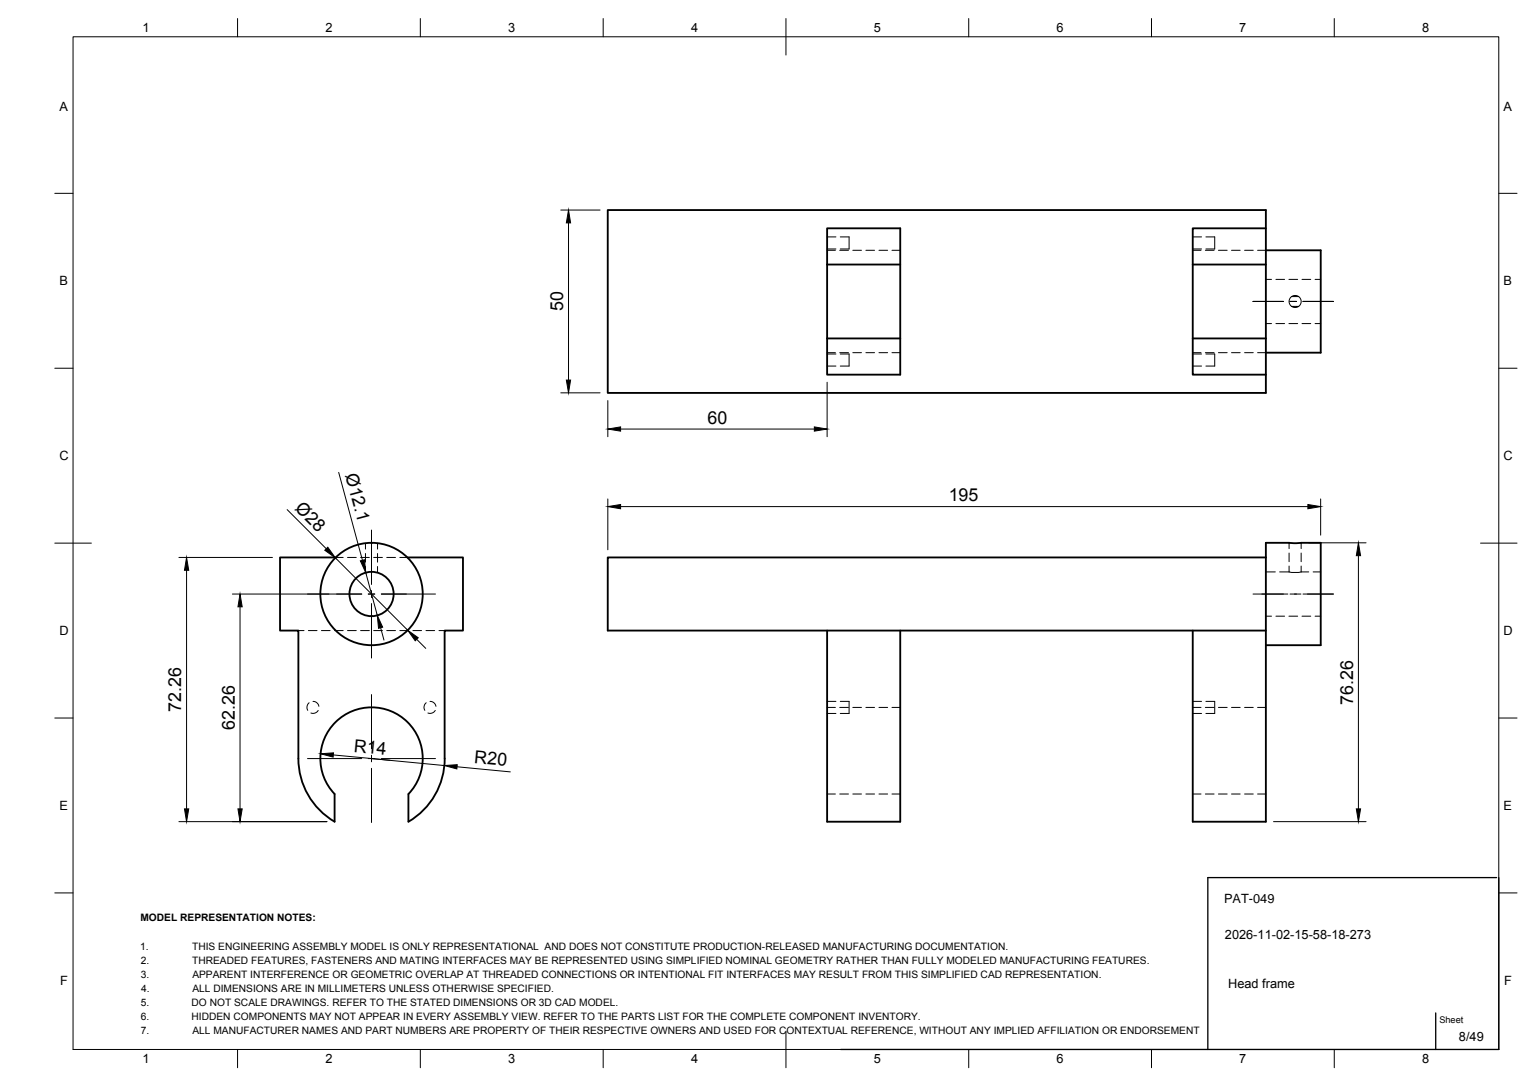
ISO-10303-21;
HEADER;
/* Generated by software containing ST-Developer
 * from STEP Tools, Inc. (www.steptools.com) 
 */

FILE_DESCRIPTION(
/* description */ ('Hand drill press frame (manual)'),
/* implementation_level */ '2;1');

FILE_NAME(
/* name */ 'Head frame.step',
/* time_stamp */ '2026-10-28T03:25:28-07:00',
/* author */ (''),
/* organization */ (''),
/* preprocessor_version */ 'ST-DEVELOPER v20.2',
/* originating_system */ 'Autodesk Translation Framework v15.17.0.0',
/* authorisation */ '');

FILE_SCHEMA (('AUTOMOTIVE_DESIGN { 1 0 10303 214 3 1 1 }'));
ENDSEC;

DATA;
#10=MECHANICAL_DESIGN_GEOMETRIC_PRESENTATION_REPRESENTATION('',(#622),#33299);
#491=B_SPLINE_CURVE_WITH_KNOTS('',3,(#18163,#18164,#18165,#18166,#18167,
#18168,#18169,#18170,#18171,#18172,#18173,#18174,#18175,#18176),
 .UNSPECIFIED.,.F.,.F.,(4,2,2,2,2,2,4),(0.598759573717645,0.624973342427789,
0.687463163426141,0.749952984424493,0.812442805422845,0.874932626421197,
0.901146395131337),.UNSPECIFIED.);
#492=B_SPLINE_CURVE_WITH_KNOTS('',3,(#18180,#18181,#18182,#18183,#18184,
#18185,#18186,#18187),.UNSPECIFIED.,.F.,.F.,(4,2,2,4),(0.249984328141498,
0.31247414913985,0.374963970138202,0.401177738848345),.UNSPECIFIED.);
#493=B_SPLINE_CURVE_WITH_KNOTS('',3,(#18191,#18192,#18193,#18194,#18195,
#18196,#18197,#18198,#18199,#18200,#18201,#18202,#18203,#18204,#18205,#18206,
#18207,#18208,#18209,#18210,#18211,#18212,#18213,#18214,#18215,#18216),
 .UNSPECIFIED.,.F.,.F.,(4,2,2,2,2,2,2,2,2,2,2,2,4),(0.,0.0622156192199746,
0.124431238439949,0.186646447577113,0.248861656714277,0.31107686585144,
0.373292074988604,0.435507694208579,0.497723313428553,0.559938932648528,
0.622154551868502,0.684369761005666,0.74658497014283),.UNSPECIFIED.);
#494=B_SPLINE_CURVE_WITH_KNOTS('',3,(#18217,#18218,#18219,#18220,#18221,
#18222,#18223,#18224,#18225,#18226),.UNSPECIFIED.,.F.,.F.,(4,2,2,2,4),(0.74658497014283,
0.808800179279993,0.871015388417157,0.933231007637132,0.995446626857106),
 .UNSPECIFIED.);
#495=B_SPLINE_CURVE_WITH_KNOTS('',3,(#18227,#18228,#18229,#18230,#18231,
#18232,#18233,#18234),.UNSPECIFIED.,.F.,.F.,(4,2,2,4),(0.098790917434652,
0.125004686144793,0.187494507143146,0.249984328141498),.UNSPECIFIED.);
#532=SHAPE_REPRESENTATION_RELATIONSHIP('SRR','None',#33491,#577);
#577=ADVANCED_BREP_SHAPE_REPRESENTATION('',(#674),#33253);
#622=STYLED_ITEM('',(#33793),#674);
#674=MANIFOLD_SOLID_BREP('Body1',#12640);
#732=FACE_BOUND('',#2075,.T.);
#733=FACE_BOUND('',#2076,.T.);
#734=FACE_BOUND('',#2090,.T.);
#735=FACE_BOUND('',#2091,.T.);
#736=FACE_BOUND('',#2095,.T.);
#737=FACE_BOUND('',#2101,.T.);
#738=FACE_BOUND('',#2103,.T.);
#739=FACE_BOUND('',#2105,.T.);
#905=PLANE('',#13233);
#906=PLANE('',#13237);
#907=PLANE('',#13238);
#908=PLANE('',#13239);
#909=PLANE('',#13240);
#910=PLANE('',#13250);
#911=PLANE('',#13251);
#912=PLANE('',#13252);
#913=PLANE('',#13256);
#914=PLANE('',#13260);
#915=PLANE('',#13261);
#916=PLANE('',#13262);
#917=PLANE('',#13263);
#918=PLANE('',#13275);
#919=PLANE('',#13276);
#920=PLANE('',#13277);
#921=PLANE('',#13278);
#922=PLANE('',#13279);
#923=PLANE('',#13283);
#924=PLANE('',#13284);
#925=PLANE('',#13291);
#926=PLANE('',#13292);
#927=PLANE('',#13293);
#928=PLANE('',#13294);
#929=PLANE('',#13295);
#930=PLANE('',#13296);
#1363=FACE_OUTER_BOUND('',#2064,.T.);
#1364=FACE_OUTER_BOUND('',#2065,.T.);
#1365=FACE_OUTER_BOUND('',#2066,.T.);
#1366=FACE_OUTER_BOUND('',#2067,.T.);
#1367=FACE_OUTER_BOUND('',#2068,.T.);
#1368=FACE_OUTER_BOUND('',#2069,.T.);
#1369=FACE_OUTER_BOUND('',#2070,.T.);
#1370=FACE_OUTER_BOUND('',#2071,.T.);
#1371=FACE_OUTER_BOUND('',#2072,.T.);
#1372=FACE_OUTER_BOUND('',#2073,.T.);
#1373=FACE_OUTER_BOUND('',#2074,.T.);
#1374=FACE_OUTER_BOUND('',#2077,.T.);
#1375=FACE_OUTER_BOUND('',#2078,.T.);
#1376=FACE_OUTER_BOUND('',#2079,.T.);
#1377=FACE_OUTER_BOUND('',#2080,.T.);
#1378=FACE_OUTER_BOUND('',#2081,.T.);
#1379=FACE_OUTER_BOUND('',#2082,.T.);
#1380=FACE_OUTER_BOUND('',#2083,.T.);
#1381=FACE_OUTER_BOUND('',#2084,.T.);
#1382=FACE_OUTER_BOUND('',#2085,.T.);
#1383=FACE_OUTER_BOUND('',#2086,.T.);
#1384=FACE_OUTER_BOUND('',#2087,.T.);
#1385=FACE_OUTER_BOUND('',#2088,.T.);
#1386=FACE_OUTER_BOUND('',#2089,.T.);
#1387=FACE_OUTER_BOUND('',#2092,.T.);
#1388=FACE_OUTER_BOUND('',#2093,.T.);
#1389=FACE_OUTER_BOUND('',#2094,.T.);
#1390=FACE_OUTER_BOUND('',#2096,.T.);
#1391=FACE_OUTER_BOUND('',#2097,.T.);
#1392=FACE_OUTER_BOUND('',#2098,.T.);
#1393=FACE_OUTER_BOUND('',#2099,.T.);
#1394=FACE_OUTER_BOUND('',#2100,.T.);
#1395=FACE_OUTER_BOUND('',#2102,.T.);
#1396=FACE_OUTER_BOUND('',#2104,.T.);
#1397=FACE_OUTER_BOUND('',#2106,.T.);
#1398=FACE_OUTER_BOUND('',#2107,.T.);
#1399=FACE_OUTER_BOUND('',#2108,.T.);
#1400=FACE_OUTER_BOUND('',#2109,.T.);
#1401=FACE_OUTER_BOUND('',#2110,.T.);
#2064=EDGE_LOOP('',(#8529,#8530,#8531,#8532));
#2065=EDGE_LOOP('',(#8533));
#2066=EDGE_LOOP('',(#8534,#8535,#8536,#8537));
#2067=EDGE_LOOP('',(#8538));
#2068=EDGE_LOOP('',(#8539,#8540,#8541,#8542));
#2069=EDGE_LOOP('',(#8543,#8544,#8545,#8546));
#2070=EDGE_LOOP('',(#8547,#8548,#8549,#8550,#8551,#8552,#8553,#8554));
#2071=EDGE_LOOP('',(#8555,#8556,#8557,#8558));
#2072=EDGE_LOOP('',(#8559,#8560,#8561,#8562));
#2073=EDGE_LOOP('',(#8563,#8564,#8565,#8566));
#2074=EDGE_LOOP('',(#8567,#8568,#8569,#8570,#8571,#8572,#8573,#8574));
#2075=EDGE_LOOP('',(#8575));
#2076=EDGE_LOOP('',(#8576));
#2077=EDGE_LOOP('',(#8577,#8578,#8579,#8580));
#2078=EDGE_LOOP('',(#8581,#8582,#8583,#8584));
#2079=EDGE_LOOP('',(#8585,#8586,#8587,#8588));
#2080=EDGE_LOOP('',(#8589));
#2081=EDGE_LOOP('',(#8590,#8591,#8592,#8593));
#2082=EDGE_LOOP('',(#8594));
#2083=EDGE_LOOP('',(#8595,#8596,#8597,#8598));
#2084=EDGE_LOOP('',(#8599,#8600,#8601,#8602));
#2085=EDGE_LOOP('',(#8603,#8604,#8605,#8606,#8607,#8608,#8609,#8610,#8611,
#8612,#8613,#8614,#8615,#8616,#8617));
#2086=EDGE_LOOP('',(#8618,#8619,#8620,#8621));
#2087=EDGE_LOOP('',(#8622,#8623,#8624,#8625));
#2088=EDGE_LOOP('',(#8626,#8627,#8628,#8629));
#2089=EDGE_LOOP('',(#8630,#8631,#8632,#8633,#8634,#8635,#8636,#8637));
#2090=EDGE_LOOP('',(#8638));
#2091=EDGE_LOOP('',(#8639));
#2092=EDGE_LOOP('',(#8640,#8641,#8642,#8643));
#2093=EDGE_LOOP('',(#8644,#8645,#8646,#8647));
#2094=EDGE_LOOP('',(#8648,#8649,#8650,#8651,#8652,#8653,#8654,#8655));
#2095=EDGE_LOOP('',(#8656,#8657,#8658,#8659));
#2096=EDGE_LOOP('',(#8660,#8661));
#2097=EDGE_LOOP('',(#8662,#8663,#8664,#8665,#8666,#8667,#8668,#8669,#8670));
#2098=EDGE_LOOP('',(#8671,#8672));
#2099=EDGE_LOOP('',(#8673,#8674));
#2100=EDGE_LOOP('',(#8675,#8676,#8677,#8678));
#2101=EDGE_LOOP('',(#8679,#8680,#8681,#8682,#8683));
#2102=EDGE_LOOP('',(#8684,#8685,#8686,#8687,#8688,#8689));
#2103=EDGE_LOOP('',(#8690,#8691));
#2104=EDGE_LOOP('',(#8692));
#2105=EDGE_LOOP('',(#8693));
#2106=EDGE_LOOP('',(#8694,#8695,#8696,#8697));
#2107=EDGE_LOOP('',(#8698,#8699,#8700,#8701,#8702,#8703));
#2108=EDGE_LOOP('',(#8704,#8705,#8706,#8707));
#2109=EDGE_LOOP('',(#8708,#8709,#8710,#8711));
#2110=EDGE_LOOP('',(#8712));
#2926=LINE('',#18014,#4091);
#2927=LINE('',#18021,#4092);
#2928=LINE('',#18027,#4093);
#2929=LINE('',#18029,#4094);
#2930=LINE('',#18031,#4095);
#2931=LINE('',#18032,#4096);
#2932=LINE('',#18036,#4097);
#2933=LINE('',#18038,#4098);
#2934=LINE('',#18040,#4099);
#2935=LINE('',#18041,#4100);
#2936=LINE('',#18046,#4101);
#2937=LINE('',#18048,#4102);
#2938=LINE('',#18050,#4103);
#2939=LINE('',#18057,#4104);
#2940=LINE('',#18062,#4105);
#2941=LINE('',#18065,#4106);
#2942=LINE('',#18067,#4107);
#2943=LINE('',#18068,#4108);
#2944=LINE('',#18070,#4109);
#2945=LINE('',#18072,#4110);
#2946=LINE('',#18077,#4111);
#2947=LINE('',#18084,#4112);
#2948=LINE('',#18090,#4113);
#2949=LINE('',#18092,#4114);
#2950=LINE('',#18094,#4115);
#2951=LINE('',#18095,#4116);
#2952=LINE('',#18099,#4117);
#2953=LINE('',#18101,#4118);
#2954=LINE('',#18103,#4119);
#2955=LINE('',#18104,#4120);
#2956=LINE('',#18109,#4121);
#2957=LINE('',#18111,#4122);
#2958=LINE('',#18113,#4123);
#2959=LINE('',#18115,#4124);
#2960=LINE('',#18121,#4125);
#2961=LINE('',#18123,#4126);
#2962=LINE('',#18125,#4127);
#2963=LINE('',#18127,#4128);
#2964=LINE('',#18134,#4129);
#2965=LINE('',#18139,#4130);
#2966=LINE('',#18142,#4131);
#2967=LINE('',#18144,#4132);
#2968=LINE('',#18145,#4133);
#2969=LINE('',#18147,#4134);
#2970=LINE('',#18149,#4135);
#2971=LINE('',#18152,#4136);
#2972=LINE('',#18154,#4137);
#2973=LINE('',#18155,#4138);
#2974=LINE('',#18159,#4139);
#2975=LINE('',#18189,#4140);
#2976=LINE('',#18236,#4141);
#2977=LINE('',#18238,#4142);
#2978=LINE('',#18244,#4143);
#2979=LINE('',#18248,#4144);
#2980=LINE('',#18253,#4145);
#2981=LINE('',#18254,#4146);
#2982=LINE('',#18257,#4147);
#2983=LINE('',#18258,#4148);
#2984=LINE('',#18260,#4149);
#4091=VECTOR('',#14497,0.165);
#4092=VECTOR('',#14506,0.165);
#4093=VECTOR('',#14513,1.);
#4094=VECTOR('',#14514,1.);
#4095=VECTOR('',#14515,1.);
#4096=VECTOR('',#14516,1.);
#4097=VECTOR('',#14519,1.);
#4098=VECTOR('',#14520,1.);
#4099=VECTOR('',#14521,1.);
#4100=VECTOR('',#14522,1.);
#4101=VECTOR('',#14527,1.);
#4102=VECTOR('',#14528,1.);
#4103=VECTOR('',#14529,1.);
#4104=VECTOR('',#14540,1.);
#4105=VECTOR('',#14547,1.);
#4106=VECTOR('',#14550,1.);
#4107=VECTOR('',#14551,1.);
#4108=VECTOR('',#14552,1.);
#4109=VECTOR('',#14555,1.);
#4110=VECTOR('',#14558,1.);
#4111=VECTOR('',#14563,0.165);
#4112=VECTOR('',#14572,0.165);
#4113=VECTOR('',#14579,1.);
#4114=VECTOR('',#14580,1.);
#4115=VECTOR('',#14581,1.);
#4116=VECTOR('',#14582,1.);
#4117=VECTOR('',#14585,1.);
#4118=VECTOR('',#14586,1.);
#4119=VECTOR('',#14587,1.);
#4120=VECTOR('',#14588,1.);
#4121=VECTOR('',#14593,1.);
#4122=VECTOR('',#14594,1.);
#4123=VECTOR('',#14595,1.);
#4124=VECTOR('',#14596,1.);
#4125=VECTOR('',#14601,1.);
#4126=VECTOR('',#14602,1.);
#4127=VECTOR('',#14603,1.);
#4128=VECTOR('',#14604,1.);
#4129=VECTOR('',#14615,1.);
#4130=VECTOR('',#14622,1.);
#4131=VECTOR('',#14625,1.);
#4132=VECTOR('',#14626,1.);
#4133=VECTOR('',#14627,1.);
#4134=VECTOR('',#14630,1.);
#4135=VECTOR('',#14633,1.);
#4136=VECTOR('',#14636,1.);
#4137=VECTOR('',#14637,1.);
#4138=VECTOR('',#14638,1.);
#4139=VECTOR('',#14641,1.);
#4140=VECTOR('',#14648,0.164999999999999);
#4141=VECTOR('',#14651,1.);
#4142=VECTOR('',#14654,1.);
#4143=VECTOR('',#14661,0.605);
#4144=VECTOR('',#14666,1.4);
#4145=VECTOR('',#14673,1.);
#4146=VECTOR('',#14674,1.);
#4147=VECTOR('',#14677,1.);
#4148=VECTOR('',#14678,1.);
#4149=VECTOR('',#14681,1.);
#5226=CIRCLE('',#13231,0.165);
#5227=CIRCLE('',#13232,0.165);
#5228=CIRCLE('',#13235,0.165);
#5229=CIRCLE('',#13236,0.165);
#5230=CIRCLE('',#13241,2.);
#5231=CIRCLE('',#13242,2.);
#5232=CIRCLE('',#13243,1.4);
#5233=CIRCLE('',#13245,1.4);
#5234=CIRCLE('',#13247,2.);
#5235=CIRCLE('',#13249,2.);
#5236=CIRCLE('',#13254,0.165);
#5237=CIRCLE('',#13255,0.165);
#5238=CIRCLE('',#13258,0.165);
#5239=CIRCLE('',#13259,0.165);
#5240=CIRCLE('',#13264,2.);
#5241=CIRCLE('',#13265,1.4);
#5242=CIRCLE('',#13266,1.4);
#5243=CIRCLE('',#13267,2.);
#5244=CIRCLE('',#13268,1.4);
#5245=CIRCLE('',#13270,1.4);
#5246=CIRCLE('',#13272,2.);
#5247=CIRCLE('',#13274,2.);
#5248=CIRCLE('',#13280,0.164999999999999);
#5249=CIRCLE('',#13282,0.164999999999999);
#5250=CIRCLE('',#13285,1.4);
#5251=CIRCLE('',#13287,0.605);
#5252=CIRCLE('',#13288,0.605);
#5253=CIRCLE('',#13290,1.4);
#5649=VERTEX_POINT('',#18011);
#5650=VERTEX_POINT('',#18013);
#5651=VERTEX_POINT('',#18018);
#5652=VERTEX_POINT('',#18020);
#5653=VERTEX_POINT('',#18025);
#5654=VERTEX_POINT('',#18026);
#5655=VERTEX_POINT('',#18028);
#5656=VERTEX_POINT('',#18030);
#5657=VERTEX_POINT('',#18034);
#5658=VERTEX_POINT('',#18035);
#5659=VERTEX_POINT('',#18037);
#5660=VERTEX_POINT('',#18039);
#5661=VERTEX_POINT('',#18043);
#5662=VERTEX_POINT('',#18045);
#5663=VERTEX_POINT('',#18047);
#5664=VERTEX_POINT('',#18049);
#5665=VERTEX_POINT('',#18056);
#5666=VERTEX_POINT('',#18060);
#5667=VERTEX_POINT('',#18064);
#5668=VERTEX_POINT('',#18066);
#5669=VERTEX_POINT('',#18074);
#5670=VERTEX_POINT('',#18076);
#5671=VERTEX_POINT('',#18081);
#5672=VERTEX_POINT('',#18083);
#5673=VERTEX_POINT('',#18088);
#5674=VERTEX_POINT('',#18089);
#5675=VERTEX_POINT('',#18091);
#5676=VERTEX_POINT('',#18093);
#5677=VERTEX_POINT('',#18097);
#5678=VERTEX_POINT('',#18098);
#5679=VERTEX_POINT('',#18100);
#5680=VERTEX_POINT('',#18102);
#5681=VERTEX_POINT('',#18106);
#5682=VERTEX_POINT('',#18108);
#5683=VERTEX_POINT('',#18110);
#5684=VERTEX_POINT('',#18112);
#5685=VERTEX_POINT('',#18114);
#5686=VERTEX_POINT('',#18116);
#5687=VERTEX_POINT('',#18118);
#5688=VERTEX_POINT('',#18120);
#5689=VERTEX_POINT('',#18122);
#5690=VERTEX_POINT('',#18124);
#5691=VERTEX_POINT('',#18126);
#5692=VERTEX_POINT('',#18133);
#5693=VERTEX_POINT('',#18137);
#5694=VERTEX_POINT('',#18141);
#5695=VERTEX_POINT('',#18143);
#5696=VERTEX_POINT('',#18151);
#5697=VERTEX_POINT('',#18153);
#5698=VERTEX_POINT('',#18157);
#5699=VERTEX_POINT('',#18158);
#5700=VERTEX_POINT('',#18162);
#5701=VERTEX_POINT('',#18177);
#5702=VERTEX_POINT('',#18179);
#5703=VERTEX_POINT('',#18188);
#5704=VERTEX_POINT('',#18190);
#5705=VERTEX_POINT('',#18241);
#5706=VERTEX_POINT('',#18243);
#5707=VERTEX_POINT('',#18247);
#5708=VERTEX_POINT('',#18252);
#5709=VERTEX_POINT('',#18256);
#6793=EDGE_CURVE('',#5649,#5649,#5226,.T.);
#6794=EDGE_CURVE('',#5649,#5650,#2926,.T.);
#6795=EDGE_CURVE('',#5650,#5650,#5227,.T.);
#6796=EDGE_CURVE('',#5651,#5651,#5228,.T.);
#6797=EDGE_CURVE('',#5651,#5652,#2927,.T.);
#6798=EDGE_CURVE('',#5652,#5652,#5229,.T.);
#6799=EDGE_CURVE('',#5653,#5654,#2928,.T.);
#6800=EDGE_CURVE('',#5655,#5653,#2929,.T.);
#6801=EDGE_CURVE('',#5656,#5655,#2930,.T.);
#6802=EDGE_CURVE('',#5654,#5656,#2931,.T.);
#6803=EDGE_CURVE('',#5657,#5658,#2932,.T.);
#6804=EDGE_CURVE('',#5659,#5657,#2933,.T.);
#6805=EDGE_CURVE('',#5660,#5659,#2934,.T.);
#6806=EDGE_CURVE('',#5658,#5660,#2935,.T.);
#6807=EDGE_CURVE('',#5661,#5653,#5230,.T.);
#6808=EDGE_CURVE('',#5662,#5661,#2936,.T.);
#6809=EDGE_CURVE('',#5663,#5662,#2937,.T.);
#6810=EDGE_CURVE('',#5664,#5663,#2938,.T.);
#6811=EDGE_CURVE('',#5658,#5664,#5231,.T.);
#6812=EDGE_CURVE('',#5660,#5655,#5232,.T.);
#6813=EDGE_CURVE('',#5656,#5659,#5233,.T.);
#6814=EDGE_CURVE('',#5664,#5665,#2939,.T.);
#6815=EDGE_CURVE('',#5657,#5665,#5234,.T.);
#6816=EDGE_CURVE('',#5666,#5654,#5235,.T.);
#6817=EDGE_CURVE('',#5661,#5666,#2940,.T.);
#6818=EDGE_CURVE('',#5665,#5667,#2941,.T.);
#6819=EDGE_CURVE('',#5668,#5667,#2942,.T.);
#6820=EDGE_CURVE('',#5668,#5666,#2943,.T.);
#6821=EDGE_CURVE('',#5667,#5663,#2944,.T.);
#6822=EDGE_CURVE('',#5662,#5668,#2945,.T.);
#6823=EDGE_CURVE('',#5669,#5669,#5236,.T.);
#6824=EDGE_CURVE('',#5669,#5670,#2946,.T.);
#6825=EDGE_CURVE('',#5670,#5670,#5237,.T.);
#6826=EDGE_CURVE('',#5671,#5671,#5238,.T.);
#6827=EDGE_CURVE('',#5671,#5672,#2947,.T.);
#6828=EDGE_CURVE('',#5672,#5672,#5239,.T.);
#6829=EDGE_CURVE('',#5673,#5674,#2948,.T.);
#6830=EDGE_CURVE('',#5675,#5673,#2949,.T.);
#6831=EDGE_CURVE('',#5676,#5675,#2950,.T.);
#6832=EDGE_CURVE('',#5674,#5676,#2951,.T.);
#6833=EDGE_CURVE('',#5677,#5678,#2952,.T.);
#6834=EDGE_CURVE('',#5679,#5677,#2953,.T.);
#6835=EDGE_CURVE('',#5680,#5679,#2954,.T.);
#6836=EDGE_CURVE('',#5678,#5680,#2955,.T.);
#6837=EDGE_CURVE('',#5681,#5673,#5240,.T.);
#6838=EDGE_CURVE('',#5682,#5681,#2956,.T.);
#6839=EDGE_CURVE('',#5683,#5682,#2957,.T.);
#6840=EDGE_CURVE('',#5684,#5683,#2958,.T.);
#6841=EDGE_CURVE('',#5685,#5684,#2959,.T.);
#6842=EDGE_CURVE('',#5685,#5686,#5241,.T.);
#6843=EDGE_CURVE('',#5686,#5687,#5242,.T.);
#6844=EDGE_CURVE('',#5688,#5687,#2960,.T.);
#6845=EDGE_CURVE('',#5689,#5688,#2961,.T.);
#6846=EDGE_CURVE('',#5690,#5689,#2962,.T.);
#6847=EDGE_CURVE('',#5691,#5690,#2963,.T.);
#6848=EDGE_CURVE('',#5678,#5691,#5243,.T.);
#6849=EDGE_CURVE('',#5680,#5675,#5244,.T.);
#6850=EDGE_CURVE('',#5676,#5679,#5245,.T.);
#6851=EDGE_CURVE('',#5691,#5692,#2964,.T.);
#6852=EDGE_CURVE('',#5677,#5692,#5246,.T.);
#6853=EDGE_CURVE('',#5693,#5674,#5247,.T.);
#6854=EDGE_CURVE('',#5681,#5693,#2965,.T.);
#6855=EDGE_CURVE('',#5692,#5694,#2966,.T.);
#6856=EDGE_CURVE('',#5695,#5694,#2967,.T.);
#6857=EDGE_CURVE('',#5695,#5693,#2968,.T.);
#6858=EDGE_CURVE('',#5682,#5695,#2969,.T.);
#6859=EDGE_CURVE('',#5694,#5690,#2970,.T.);
#6860=EDGE_CURVE('',#5689,#5696,#2971,.T.);
#6861=EDGE_CURVE('',#5697,#5696,#2972,.T.);
#6862=EDGE_CURVE('',#5683,#5697,#2973,.T.);
#6863=EDGE_CURVE('',#5698,#5699,#2974,.T.);
#6864=EDGE_CURVE('',#5698,#5699,#5248,.T.);
#6865=EDGE_CURVE('',#5700,#5698,#491,.T.);
#6866=EDGE_CURVE('',#5701,#5700,#5249,.T.);
#6867=EDGE_CURVE('',#5702,#5701,#492,.T.);
#6868=EDGE_CURVE('',#5702,#5703,#2975,.T.);
#6869=EDGE_CURVE('',#5704,#5703,#493,.T.);
#6870=EDGE_CURVE('',#5703,#5704,#494,.T.);
#6871=EDGE_CURVE('',#5699,#5702,#495,.T.);
#6872=EDGE_CURVE('',#5701,#5700,#2976,.T.);
#6873=EDGE_CURVE('',#5687,#5685,#2977,.T.);
#6874=EDGE_CURVE('',#5687,#5685,#5250,.T.);
#6875=EDGE_CURVE('',#5705,#5705,#5251,.T.);
#6876=EDGE_CURVE('',#5705,#5706,#2978,.T.);
#6877=EDGE_CURVE('',#5706,#5706,#5252,.T.);
#6878=EDGE_CURVE('',#5686,#5707,#2979,.T.);
#6879=EDGE_CURVE('',#5707,#5707,#5253,.T.);
#6880=EDGE_CURVE('',#5708,#5697,#2980,.T.);
#6881=EDGE_CURVE('',#5684,#5708,#2981,.T.);
#6882=EDGE_CURVE('',#5709,#5708,#2982,.T.);
#6883=EDGE_CURVE('',#5688,#5709,#2983,.T.);
#6884=EDGE_CURVE('',#5696,#5709,#2984,.T.);
#8529=ORIENTED_EDGE('',*,*,#6793,.F.);
#8530=ORIENTED_EDGE('',*,*,#6794,.T.);
#8531=ORIENTED_EDGE('',*,*,#6795,.F.);
#8532=ORIENTED_EDGE('',*,*,#6794,.F.);
#8533=ORIENTED_EDGE('',*,*,#6793,.T.);
#8534=ORIENTED_EDGE('',*,*,#6796,.F.);
#8535=ORIENTED_EDGE('',*,*,#6797,.T.);
#8536=ORIENTED_EDGE('',*,*,#6798,.F.);
#8537=ORIENTED_EDGE('',*,*,#6797,.F.);
#8538=ORIENTED_EDGE('',*,*,#6796,.T.);
#8539=ORIENTED_EDGE('',*,*,#6799,.F.);
#8540=ORIENTED_EDGE('',*,*,#6800,.F.);
#8541=ORIENTED_EDGE('',*,*,#6801,.F.);
#8542=ORIENTED_EDGE('',*,*,#6802,.F.);
#8543=ORIENTED_EDGE('',*,*,#6803,.F.);
#8544=ORIENTED_EDGE('',*,*,#6804,.F.);
#8545=ORIENTED_EDGE('',*,*,#6805,.F.);
#8546=ORIENTED_EDGE('',*,*,#6806,.F.);
#8547=ORIENTED_EDGE('',*,*,#6800,.T.);
#8548=ORIENTED_EDGE('',*,*,#6807,.F.);
#8549=ORIENTED_EDGE('',*,*,#6808,.F.);
#8550=ORIENTED_EDGE('',*,*,#6809,.F.);
#8551=ORIENTED_EDGE('',*,*,#6810,.F.);
#8552=ORIENTED_EDGE('',*,*,#6811,.F.);
#8553=ORIENTED_EDGE('',*,*,#6806,.T.);
#8554=ORIENTED_EDGE('',*,*,#6812,.T.);
#8555=ORIENTED_EDGE('',*,*,#6801,.T.);
#8556=ORIENTED_EDGE('',*,*,#6812,.F.);
#8557=ORIENTED_EDGE('',*,*,#6805,.T.);
#8558=ORIENTED_EDGE('',*,*,#6813,.F.);
#8559=ORIENTED_EDGE('',*,*,#6803,.T.);
#8560=ORIENTED_EDGE('',*,*,#6811,.T.);
#8561=ORIENTED_EDGE('',*,*,#6814,.T.);
#8562=ORIENTED_EDGE('',*,*,#6815,.F.);
#8563=ORIENTED_EDGE('',*,*,#6799,.T.);
#8564=ORIENTED_EDGE('',*,*,#6816,.F.);
#8565=ORIENTED_EDGE('',*,*,#6817,.F.);
#8566=ORIENTED_EDGE('',*,*,#6807,.T.);
#8567=ORIENTED_EDGE('',*,*,#6802,.T.);
#8568=ORIENTED_EDGE('',*,*,#6813,.T.);
#8569=ORIENTED_EDGE('',*,*,#6804,.T.);
#8570=ORIENTED_EDGE('',*,*,#6815,.T.);
#8571=ORIENTED_EDGE('',*,*,#6818,.T.);
#8572=ORIENTED_EDGE('',*,*,#6819,.F.);
#8573=ORIENTED_EDGE('',*,*,#6820,.T.);
#8574=ORIENTED_EDGE('',*,*,#6816,.T.);
#8575=ORIENTED_EDGE('',*,*,#6795,.T.);
#8576=ORIENTED_EDGE('',*,*,#6798,.T.);
#8577=ORIENTED_EDGE('',*,*,#6821,.F.);
#8578=ORIENTED_EDGE('',*,*,#6818,.F.);
#8579=ORIENTED_EDGE('',*,*,#6814,.F.);
#8580=ORIENTED_EDGE('',*,*,#6810,.T.);
#8581=ORIENTED_EDGE('',*,*,#6822,.F.);
#8582=ORIENTED_EDGE('',*,*,#6808,.T.);
#8583=ORIENTED_EDGE('',*,*,#6817,.T.);
#8584=ORIENTED_EDGE('',*,*,#6820,.F.);
#8585=ORIENTED_EDGE('',*,*,#6823,.F.);
#8586=ORIENTED_EDGE('',*,*,#6824,.T.);
#8587=ORIENTED_EDGE('',*,*,#6825,.F.);
#8588=ORIENTED_EDGE('',*,*,#6824,.F.);
#8589=ORIENTED_EDGE('',*,*,#6823,.T.);
#8590=ORIENTED_EDGE('',*,*,#6826,.F.);
#8591=ORIENTED_EDGE('',*,*,#6827,.T.);
#8592=ORIENTED_EDGE('',*,*,#6828,.F.);
#8593=ORIENTED_EDGE('',*,*,#6827,.F.);
#8594=ORIENTED_EDGE('',*,*,#6826,.T.);
#8595=ORIENTED_EDGE('',*,*,#6829,.F.);
#8596=ORIENTED_EDGE('',*,*,#6830,.F.);
#8597=ORIENTED_EDGE('',*,*,#6831,.F.);
#8598=ORIENTED_EDGE('',*,*,#6832,.F.);
#8599=ORIENTED_EDGE('',*,*,#6833,.F.);
#8600=ORIENTED_EDGE('',*,*,#6834,.F.);
#8601=ORIENTED_EDGE('',*,*,#6835,.F.);
#8602=ORIENTED_EDGE('',*,*,#6836,.F.);
#8603=ORIENTED_EDGE('',*,*,#6830,.T.);
#8604=ORIENTED_EDGE('',*,*,#6837,.F.);
#8605=ORIENTED_EDGE('',*,*,#6838,.F.);
#8606=ORIENTED_EDGE('',*,*,#6839,.F.);
#8607=ORIENTED_EDGE('',*,*,#6840,.F.);
#8608=ORIENTED_EDGE('',*,*,#6841,.F.);
#8609=ORIENTED_EDGE('',*,*,#6842,.T.);
#8610=ORIENTED_EDGE('',*,*,#6843,.T.);
#8611=ORIENTED_EDGE('',*,*,#6844,.F.);
#8612=ORIENTED_EDGE('',*,*,#6845,.F.);
#8613=ORIENTED_EDGE('',*,*,#6846,.F.);
#8614=ORIENTED_EDGE('',*,*,#6847,.F.);
#8615=ORIENTED_EDGE('',*,*,#6848,.F.);
#8616=ORIENTED_EDGE('',*,*,#6836,.T.);
#8617=ORIENTED_EDGE('',*,*,#6849,.T.);
#8618=ORIENTED_EDGE('',*,*,#6831,.T.);
#8619=ORIENTED_EDGE('',*,*,#6849,.F.);
#8620=ORIENTED_EDGE('',*,*,#6835,.T.);
#8621=ORIENTED_EDGE('',*,*,#6850,.F.);
#8622=ORIENTED_EDGE('',*,*,#6833,.T.);
#8623=ORIENTED_EDGE('',*,*,#6848,.T.);
#8624=ORIENTED_EDGE('',*,*,#6851,.T.);
#8625=ORIENTED_EDGE('',*,*,#6852,.F.);
#8626=ORIENTED_EDGE('',*,*,#6829,.T.);
#8627=ORIENTED_EDGE('',*,*,#6853,.F.);
#8628=ORIENTED_EDGE('',*,*,#6854,.F.);
#8629=ORIENTED_EDGE('',*,*,#6837,.T.);
#8630=ORIENTED_EDGE('',*,*,#6832,.T.);
#8631=ORIENTED_EDGE('',*,*,#6850,.T.);
#8632=ORIENTED_EDGE('',*,*,#6834,.T.);
#8633=ORIENTED_EDGE('',*,*,#6852,.T.);
#8634=ORIENTED_EDGE('',*,*,#6855,.T.);
#8635=ORIENTED_EDGE('',*,*,#6856,.F.);
#8636=ORIENTED_EDGE('',*,*,#6857,.T.);
#8637=ORIENTED_EDGE('',*,*,#6853,.T.);
#8638=ORIENTED_EDGE('',*,*,#6825,.T.);
#8639=ORIENTED_EDGE('',*,*,#6828,.T.);
#8640=ORIENTED_EDGE('',*,*,#6858,.F.);
#8641=ORIENTED_EDGE('',*,*,#6838,.T.);
#8642=ORIENTED_EDGE('',*,*,#6854,.T.);
#8643=ORIENTED_EDGE('',*,*,#6857,.F.);
#8644=ORIENTED_EDGE('',*,*,#6859,.F.);
#8645=ORIENTED_EDGE('',*,*,#6855,.F.);
#8646=ORIENTED_EDGE('',*,*,#6851,.F.);
#8647=ORIENTED_EDGE('',*,*,#6847,.T.);
#8648=ORIENTED_EDGE('',*,*,#6858,.T.);
#8649=ORIENTED_EDGE('',*,*,#6856,.T.);
#8650=ORIENTED_EDGE('',*,*,#6859,.T.);
#8651=ORIENTED_EDGE('',*,*,#6846,.T.);
#8652=ORIENTED_EDGE('',*,*,#6860,.T.);
#8653=ORIENTED_EDGE('',*,*,#6861,.F.);
#8654=ORIENTED_EDGE('',*,*,#6862,.F.);
#8655=ORIENTED_EDGE('',*,*,#6839,.T.);
#8656=ORIENTED_EDGE('',*,*,#6821,.T.);
#8657=ORIENTED_EDGE('',*,*,#6809,.T.);
#8658=ORIENTED_EDGE('',*,*,#6822,.T.);
#8659=ORIENTED_EDGE('',*,*,#6819,.T.);
#8660=ORIENTED_EDGE('',*,*,#6863,.F.);
#8661=ORIENTED_EDGE('',*,*,#6864,.T.);
#8662=ORIENTED_EDGE('',*,*,#6865,.F.);
#8663=ORIENTED_EDGE('',*,*,#6866,.F.);
#8664=ORIENTED_EDGE('',*,*,#6867,.F.);
#8665=ORIENTED_EDGE('',*,*,#6868,.T.);
#8666=ORIENTED_EDGE('',*,*,#6869,.F.);
#8667=ORIENTED_EDGE('',*,*,#6870,.F.);
#8668=ORIENTED_EDGE('',*,*,#6868,.F.);
#8669=ORIENTED_EDGE('',*,*,#6871,.F.);
#8670=ORIENTED_EDGE('',*,*,#6864,.F.);
#8671=ORIENTED_EDGE('',*,*,#6872,.F.);
#8672=ORIENTED_EDGE('',*,*,#6866,.T.);
#8673=ORIENTED_EDGE('',*,*,#6873,.F.);
#8674=ORIENTED_EDGE('',*,*,#6874,.T.);
#8675=ORIENTED_EDGE('',*,*,#6875,.F.);
#8676=ORIENTED_EDGE('',*,*,#6876,.T.);
#8677=ORIENTED_EDGE('',*,*,#6877,.T.);
#8678=ORIENTED_EDGE('',*,*,#6876,.F.);
#8679=ORIENTED_EDGE('',*,*,#6871,.T.);
#8680=ORIENTED_EDGE('',*,*,#6867,.T.);
#8681=ORIENTED_EDGE('',*,*,#6872,.T.);
#8682=ORIENTED_EDGE('',*,*,#6865,.T.);
#8683=ORIENTED_EDGE('',*,*,#6863,.T.);
#8684=ORIENTED_EDGE('',*,*,#6842,.F.);
#8685=ORIENTED_EDGE('',*,*,#6874,.F.);
#8686=ORIENTED_EDGE('',*,*,#6843,.F.);
#8687=ORIENTED_EDGE('',*,*,#6878,.T.);
#8688=ORIENTED_EDGE('',*,*,#6879,.T.);
#8689=ORIENTED_EDGE('',*,*,#6878,.F.);
#8690=ORIENTED_EDGE('',*,*,#6869,.T.);
#8691=ORIENTED_EDGE('',*,*,#6870,.T.);
#8692=ORIENTED_EDGE('',*,*,#6879,.F.);
#8693=ORIENTED_EDGE('',*,*,#6877,.F.);
#8694=ORIENTED_EDGE('',*,*,#6840,.T.);
#8695=ORIENTED_EDGE('',*,*,#6862,.T.);
#8696=ORIENTED_EDGE('',*,*,#6880,.F.);
#8697=ORIENTED_EDGE('',*,*,#6881,.F.);
#8698=ORIENTED_EDGE('',*,*,#6841,.T.);
#8699=ORIENTED_EDGE('',*,*,#6881,.T.);
#8700=ORIENTED_EDGE('',*,*,#6882,.F.);
#8701=ORIENTED_EDGE('',*,*,#6883,.F.);
#8702=ORIENTED_EDGE('',*,*,#6844,.T.);
#8703=ORIENTED_EDGE('',*,*,#6873,.T.);
#8704=ORIENTED_EDGE('',*,*,#6845,.T.);
#8705=ORIENTED_EDGE('',*,*,#6883,.T.);
#8706=ORIENTED_EDGE('',*,*,#6884,.F.);
#8707=ORIENTED_EDGE('',*,*,#6860,.F.);
#8708=ORIENTED_EDGE('',*,*,#6861,.T.);
#8709=ORIENTED_EDGE('',*,*,#6884,.T.);
#8710=ORIENTED_EDGE('',*,*,#6882,.T.);
#8711=ORIENTED_EDGE('',*,*,#6880,.T.);
#8712=ORIENTED_EDGE('',*,*,#6875,.T.);
#11791=CYLINDRICAL_SURFACE('',#13230,0.165);
#11792=CYLINDRICAL_SURFACE('',#13234,0.165);
#11793=CYLINDRICAL_SURFACE('',#13244,1.4);
#11794=CYLINDRICAL_SURFACE('',#13246,2.);
#11795=CYLINDRICAL_SURFACE('',#13248,2.);
#11796=CYLINDRICAL_SURFACE('',#13253,0.165);
#11797=CYLINDRICAL_SURFACE('',#13257,0.165);
#11798=CYLINDRICAL_SURFACE('',#13269,1.4);
#11799=CYLINDRICAL_SURFACE('',#13271,2.);
#11800=CYLINDRICAL_SURFACE('',#13273,2.);
#11801=CYLINDRICAL_SURFACE('',#13281,0.164999999999999);
#11802=CYLINDRICAL_SURFACE('',#13286,0.605);
#11803=CYLINDRICAL_SURFACE('',#13289,1.4);
#11972=ADVANCED_FACE('',(#1363),#11791,.F.);
#11973=ADVANCED_FACE('',(#1364),#905,.T.);
#11974=ADVANCED_FACE('',(#1365),#11792,.F.);
#11975=ADVANCED_FACE('',(#1366),#906,.T.);
#11976=ADVANCED_FACE('',(#1367),#907,.F.);
#11977=ADVANCED_FACE('',(#1368),#908,.F.);
#11978=ADVANCED_FACE('',(#1369),#909,.F.);
#11979=ADVANCED_FACE('',(#1370),#11793,.F.);
#11980=ADVANCED_FACE('',(#1371),#11794,.T.);
#11981=ADVANCED_FACE('',(#1372),#11795,.T.);
#11982=ADVANCED_FACE('',(#1373,#732,#733),#910,.T.);
#11983=ADVANCED_FACE('',(#1374),#911,.T.);
#11984=ADVANCED_FACE('',(#1375),#912,.T.);
#11985=ADVANCED_FACE('',(#1376),#11796,.F.);
#11986=ADVANCED_FACE('',(#1377),#913,.T.);
#11987=ADVANCED_FACE('',(#1378),#11797,.F.);
#11988=ADVANCED_FACE('',(#1379),#914,.T.);
#11989=ADVANCED_FACE('',(#1380),#915,.F.);
#11990=ADVANCED_FACE('',(#1381),#916,.F.);
#11991=ADVANCED_FACE('',(#1382),#917,.F.);
#11992=ADVANCED_FACE('',(#1383),#11798,.F.);
#11993=ADVANCED_FACE('',(#1384),#11799,.T.);
#11994=ADVANCED_FACE('',(#1385),#11800,.T.);
#11995=ADVANCED_FACE('',(#1386,#734,#735),#918,.T.);
#11996=ADVANCED_FACE('',(#1387),#919,.T.);
#11997=ADVANCED_FACE('',(#1388),#920,.T.);
#11998=ADVANCED_FACE('',(#1389,#736),#921,.T.);
#11999=ADVANCED_FACE('',(#1390),#922,.T.);
#12000=ADVANCED_FACE('',(#1391),#11801,.F.);
#12001=ADVANCED_FACE('',(#1392),#923,.T.);
#12002=ADVANCED_FACE('',(#1393),#924,.T.);
#12003=ADVANCED_FACE('',(#1394,#737),#11802,.F.);
#12004=ADVANCED_FACE('',(#1395,#738),#11803,.T.);
#12005=ADVANCED_FACE('',(#1396,#739),#925,.F.);
#12006=ADVANCED_FACE('',(#1397),#926,.T.);
#12007=ADVANCED_FACE('',(#1398),#927,.T.);
#12008=ADVANCED_FACE('',(#1399),#928,.T.);
#12009=ADVANCED_FACE('',(#1400),#929,.T.);
#12010=ADVANCED_FACE('',(#1401),#930,.F.);
#12640=CLOSED_SHELL('',(#11972,#11973,#11974,#11975,#11976,#11977,#11978,
#11979,#11980,#11981,#11982,#11983,#11984,#11985,#11986,#11987,#11988,#11989,
#11990,#11991,#11992,#11993,#11994,#11995,#11996,#11997,#11998,#11999,#12000,
#12001,#12002,#12003,#12004,#12005,#12006,#12007,#12008,#12009,#12010));
#13229=AXIS2_PLACEMENT_3D('',#18009,#14491,#14492);
#13230=AXIS2_PLACEMENT_3D('',#18010,#14493,#14494);
#13231=AXIS2_PLACEMENT_3D('',#18012,#14495,#14496);
#13232=AXIS2_PLACEMENT_3D('',#18015,#14498,#14499);
#13233=AXIS2_PLACEMENT_3D('',#18016,#14500,#14501);
#13234=AXIS2_PLACEMENT_3D('',#18017,#14502,#14503);
#13235=AXIS2_PLACEMENT_3D('',#18019,#14504,#14505);
#13236=AXIS2_PLACEMENT_3D('',#18022,#14507,#14508);
#13237=AXIS2_PLACEMENT_3D('',#18023,#14509,#14510);
#13238=AXIS2_PLACEMENT_3D('',#18024,#14511,#14512);
#13239=AXIS2_PLACEMENT_3D('',#18033,#14517,#14518);
#13240=AXIS2_PLACEMENT_3D('',#18042,#14523,#14524);
#13241=AXIS2_PLACEMENT_3D('',#18044,#14525,#14526);
#13242=AXIS2_PLACEMENT_3D('',#18051,#14530,#14531);
#13243=AXIS2_PLACEMENT_3D('',#18052,#14532,#14533);
#13244=AXIS2_PLACEMENT_3D('',#18053,#14534,#14535);
#13245=AXIS2_PLACEMENT_3D('',#18054,#14536,#14537);
#13246=AXIS2_PLACEMENT_3D('',#18055,#14538,#14539);
#13247=AXIS2_PLACEMENT_3D('',#18058,#14541,#14542);
#13248=AXIS2_PLACEMENT_3D('',#18059,#14543,#14544);
#13249=AXIS2_PLACEMENT_3D('',#18061,#14545,#14546);
#13250=AXIS2_PLACEMENT_3D('',#18063,#14548,#14549);
#13251=AXIS2_PLACEMENT_3D('',#18069,#14553,#14554);
#13252=AXIS2_PLACEMENT_3D('',#18071,#14556,#14557);
#13253=AXIS2_PLACEMENT_3D('',#18073,#14559,#14560);
#13254=AXIS2_PLACEMENT_3D('',#18075,#14561,#14562);
#13255=AXIS2_PLACEMENT_3D('',#18078,#14564,#14565);
#13256=AXIS2_PLACEMENT_3D('',#18079,#14566,#14567);
#13257=AXIS2_PLACEMENT_3D('',#18080,#14568,#14569);
#13258=AXIS2_PLACEMENT_3D('',#18082,#14570,#14571);
#13259=AXIS2_PLACEMENT_3D('',#18085,#14573,#14574);
#13260=AXIS2_PLACEMENT_3D('',#18086,#14575,#14576);
#13261=AXIS2_PLACEMENT_3D('',#18087,#14577,#14578);
#13262=AXIS2_PLACEMENT_3D('',#18096,#14583,#14584);
#13263=AXIS2_PLACEMENT_3D('',#18105,#14589,#14590);
#13264=AXIS2_PLACEMENT_3D('',#18107,#14591,#14592);
#13265=AXIS2_PLACEMENT_3D('',#18117,#14597,#14598);
#13266=AXIS2_PLACEMENT_3D('',#18119,#14599,#14600);
#13267=AXIS2_PLACEMENT_3D('',#18128,#14605,#14606);
#13268=AXIS2_PLACEMENT_3D('',#18129,#14607,#14608);
#13269=AXIS2_PLACEMENT_3D('',#18130,#14609,#14610);
#13270=AXIS2_PLACEMENT_3D('',#18131,#14611,#14612);
#13271=AXIS2_PLACEMENT_3D('',#18132,#14613,#14614);
#13272=AXIS2_PLACEMENT_3D('',#18135,#14616,#14617);
#13273=AXIS2_PLACEMENT_3D('',#18136,#14618,#14619);
#13274=AXIS2_PLACEMENT_3D('',#18138,#14620,#14621);
#13275=AXIS2_PLACEMENT_3D('',#18140,#14623,#14624);
#13276=AXIS2_PLACEMENT_3D('',#18146,#14628,#14629);
#13277=AXIS2_PLACEMENT_3D('',#18148,#14631,#14632);
#13278=AXIS2_PLACEMENT_3D('',#18150,#14634,#14635);
#13279=AXIS2_PLACEMENT_3D('',#18156,#14639,#14640);
#13280=AXIS2_PLACEMENT_3D('',#18160,#14642,#14643);
#13281=AXIS2_PLACEMENT_3D('',#18161,#14644,#14645);
#13282=AXIS2_PLACEMENT_3D('',#18178,#14646,#14647);
#13283=AXIS2_PLACEMENT_3D('',#18235,#14649,#14650);
#13284=AXIS2_PLACEMENT_3D('',#18237,#14652,#14653);
#13285=AXIS2_PLACEMENT_3D('',#18239,#14655,#14656);
#13286=AXIS2_PLACEMENT_3D('',#18240,#14657,#14658);
#13287=AXIS2_PLACEMENT_3D('',#18242,#14659,#14660);
#13288=AXIS2_PLACEMENT_3D('',#18245,#14662,#14663);
#13289=AXIS2_PLACEMENT_3D('',#18246,#14664,#14665);
#13290=AXIS2_PLACEMENT_3D('',#18249,#14667,#14668);
#13291=AXIS2_PLACEMENT_3D('',#18250,#14669,#14670);
#13292=AXIS2_PLACEMENT_3D('',#18251,#14671,#14672);
#13293=AXIS2_PLACEMENT_3D('',#18255,#14675,#14676);
#13294=AXIS2_PLACEMENT_3D('',#18259,#14679,#14680);
#13295=AXIS2_PLACEMENT_3D('',#18261,#14682,#14683);
#13296=AXIS2_PLACEMENT_3D('',#18262,#14684,#14685);
#14491=DIRECTION('axis',(0.,0.,1.));
#14492=DIRECTION('refdir',(1.,0.,0.));
#14493=DIRECTION('center_axis',(0.,0.,1.));
#14494=DIRECTION('ref_axis',(1.,0.,0.));
#14495=DIRECTION('center_axis',(0.,0.,1.));
#14496=DIRECTION('ref_axis',(1.,0.,0.));
#14497=DIRECTION('',(0.,0.,1.));
#14498=DIRECTION('center_axis',(0.,0.,-1.));
#14499=DIRECTION('ref_axis',(1.,0.,0.));
#14500=DIRECTION('center_axis',(0.,0.,1.));
#14501=DIRECTION('ref_axis',(1.,0.,0.));
#14502=DIRECTION('center_axis',(0.,0.,1.));
#14503=DIRECTION('ref_axis',(1.,0.,0.));
#14504=DIRECTION('center_axis',(0.,0.,1.));
#14505=DIRECTION('ref_axis',(1.,0.,0.));
#14506=DIRECTION('',(0.,0.,1.));
#14507=DIRECTION('center_axis',(0.,0.,-1.));
#14508=DIRECTION('ref_axis',(1.,0.,0.));
#14509=DIRECTION('center_axis',(0.,0.,1.));
#14510=DIRECTION('ref_axis',(1.,0.,0.));
#14511=DIRECTION('center_axis',(0.,1.,0.));
#14512=DIRECTION('ref_axis',(-1.,0.,0.));
#14513=DIRECTION('',(0.,0.,1.));
#14514=DIRECTION('',(-1.,0.,0.));
#14515=DIRECTION('',(0.,0.,-1.));
#14516=DIRECTION('',(1.,0.,0.));
#14517=DIRECTION('center_axis',(0.,-1.,0.));
#14518=DIRECTION('ref_axis',(1.,0.,0.));
#14519=DIRECTION('',(0.,0.,-1.));
#14520=DIRECTION('',(-1.,0.,0.));
#14521=DIRECTION('',(0.,0.,1.));
#14522=DIRECTION('',(1.,0.,0.));
#14523=DIRECTION('center_axis',(0.,0.,1.));
#14524=DIRECTION('ref_axis',(1.,0.,0.));
#14525=DIRECTION('center_axis',(0.,0.,1.));
#14526=DIRECTION('ref_axis',(1.,0.,0.));
#14527=DIRECTION('',(-1.,0.,0.));
#14528=DIRECTION('',(0.,1.,0.));
#14529=DIRECTION('',(1.,0.,0.));
#14530=DIRECTION('center_axis',(0.,0.,1.));
#14531=DIRECTION('ref_axis',(1.,0.,0.));
#14532=DIRECTION('center_axis',(0.,0.,1.));
#14533=DIRECTION('ref_axis',(1.,0.,0.));
#14534=DIRECTION('center_axis',(0.,0.,1.));
#14535=DIRECTION('ref_axis',(1.,0.,0.));
#14536=DIRECTION('center_axis',(0.,0.,-1.));
#14537=DIRECTION('ref_axis',(1.,0.,0.));
#14538=DIRECTION('center_axis',(0.,0.,1.));
#14539=DIRECTION('ref_axis',(1.,0.,0.));
#14540=DIRECTION('',(0.,0.,1.));
#14541=DIRECTION('center_axis',(0.,0.,1.));
#14542=DIRECTION('ref_axis',(1.,0.,0.));
#14543=DIRECTION('center_axis',(0.,0.,1.));
#14544=DIRECTION('ref_axis',(1.,0.,0.));
#14545=DIRECTION('center_axis',(0.,0.,1.));
#14546=DIRECTION('ref_axis',(1.,0.,0.));
#14547=DIRECTION('',(0.,0.,1.));
#14548=DIRECTION('center_axis',(0.,0.,1.));
#14549=DIRECTION('ref_axis',(1.,0.,0.));
#14550=DIRECTION('',(1.,0.,0.));
#14551=DIRECTION('',(0.,-1.,0.));
#14552=DIRECTION('',(-1.,0.,0.));
#14553=DIRECTION('center_axis',(0.,-1.,0.));
#14554=DIRECTION('ref_axis',(1.,0.,0.));
#14555=DIRECTION('',(0.,0.,-1.));
#14556=DIRECTION('center_axis',(0.,1.,0.));
#14557=DIRECTION('ref_axis',(-1.,0.,0.));
#14558=DIRECTION('',(0.,0.,1.));
#14559=DIRECTION('center_axis',(0.,0.,1.));
#14560=DIRECTION('ref_axis',(1.,0.,0.));
#14561=DIRECTION('center_axis',(0.,0.,1.));
#14562=DIRECTION('ref_axis',(1.,0.,0.));
#14563=DIRECTION('',(0.,0.,1.));
#14564=DIRECTION('center_axis',(0.,0.,-1.));
#14565=DIRECTION('ref_axis',(1.,0.,0.));
#14566=DIRECTION('center_axis',(0.,0.,1.));
#14567=DIRECTION('ref_axis',(1.,0.,0.));
#14568=DIRECTION('center_axis',(0.,0.,1.));
#14569=DIRECTION('ref_axis',(1.,0.,0.));
#14570=DIRECTION('center_axis',(0.,0.,1.));
#14571=DIRECTION('ref_axis',(1.,0.,0.));
#14572=DIRECTION('',(0.,0.,1.));
#14573=DIRECTION('center_axis',(0.,0.,-1.));
#14574=DIRECTION('ref_axis',(1.,0.,0.));
#14575=DIRECTION('center_axis',(0.,0.,1.));
#14576=DIRECTION('ref_axis',(1.,0.,0.));
#14577=DIRECTION('center_axis',(0.,1.,0.));
#14578=DIRECTION('ref_axis',(-1.,0.,0.));
#14579=DIRECTION('',(0.,0.,1.));
#14580=DIRECTION('',(-1.,0.,0.));
#14581=DIRECTION('',(0.,0.,-1.));
#14582=DIRECTION('',(1.,0.,0.));
#14583=DIRECTION('center_axis',(0.,-1.,0.));
#14584=DIRECTION('ref_axis',(1.,0.,0.));
#14585=DIRECTION('',(0.,0.,-1.));
#14586=DIRECTION('',(-1.,0.,0.));
#14587=DIRECTION('',(0.,0.,1.));
#14588=DIRECTION('',(1.,0.,0.));
#14589=DIRECTION('center_axis',(0.,0.,1.));
#14590=DIRECTION('ref_axis',(1.,0.,0.));
#14591=DIRECTION('center_axis',(0.,0.,1.));
#14592=DIRECTION('ref_axis',(1.,0.,0.));
#14593=DIRECTION('',(-1.,0.,0.));
#14594=DIRECTION('',(0.,-1.,0.));
#14595=DIRECTION('',(-1.,0.,0.));
#14596=DIRECTION('',(0.,1.,0.));
#14597=DIRECTION('center_axis',(0.,0.,1.));
#14598=DIRECTION('ref_axis',(1.,0.,0.));
#14599=DIRECTION('center_axis',(0.,0.,1.));
#14600=DIRECTION('ref_axis',(1.,0.,0.));
#14601=DIRECTION('',(0.,1.,0.));
#14602=DIRECTION('',(1.,0.,0.));
#14603=DIRECTION('',(0.,-1.,0.));
#14604=DIRECTION('',(1.,0.,0.));
#14605=DIRECTION('center_axis',(0.,0.,1.));
#14606=DIRECTION('ref_axis',(1.,0.,0.));
#14607=DIRECTION('center_axis',(0.,0.,1.));
#14608=DIRECTION('ref_axis',(1.,0.,0.));
#14609=DIRECTION('center_axis',(0.,0.,1.));
#14610=DIRECTION('ref_axis',(1.,0.,0.));
#14611=DIRECTION('center_axis',(0.,0.,-1.));
#14612=DIRECTION('ref_axis',(1.,0.,0.));
#14613=DIRECTION('center_axis',(0.,0.,1.));
#14614=DIRECTION('ref_axis',(1.,0.,0.));
#14615=DIRECTION('',(0.,0.,1.));
#14616=DIRECTION('center_axis',(0.,0.,1.));
#14617=DIRECTION('ref_axis',(1.,0.,0.));
#14618=DIRECTION('center_axis',(0.,0.,1.));
#14619=DIRECTION('ref_axis',(1.,0.,0.));
#14620=DIRECTION('center_axis',(0.,0.,1.));
#14621=DIRECTION('ref_axis',(1.,0.,0.));
#14622=DIRECTION('',(0.,0.,1.));
#14623=DIRECTION('center_axis',(0.,0.,1.));
#14624=DIRECTION('ref_axis',(1.,0.,0.));
#14625=DIRECTION('',(1.,0.,0.));
#14626=DIRECTION('',(0.,-1.,0.));
#14627=DIRECTION('',(-1.,0.,0.));
#14628=DIRECTION('center_axis',(0.,1.,0.));
#14629=DIRECTION('ref_axis',(-1.,0.,0.));
#14630=DIRECTION('',(0.,0.,1.));
#14631=DIRECTION('center_axis',(0.,-1.,0.));
#14632=DIRECTION('ref_axis',(1.,0.,0.));
#14633=DIRECTION('',(0.,0.,-1.));
#14634=DIRECTION('center_axis',(-1.,0.,0.));
#14635=DIRECTION('ref_axis',(0.,-1.,0.));
#14636=DIRECTION('',(0.,0.,1.));
#14637=DIRECTION('',(0.,-1.,0.));
#14638=DIRECTION('',(0.,0.,1.));
#14639=DIRECTION('center_axis',(1.,0.,0.));
#14640=DIRECTION('ref_axis',(0.,0.,-1.));
#14641=DIRECTION('',(0.,0.,1.));
#14642=DIRECTION('center_axis',(1.,0.,0.));
#14643=DIRECTION('ref_axis',(0.,0.,-1.));
#14644=DIRECTION('center_axis',(1.,0.,0.));
#14645=DIRECTION('ref_axis',(0.,0.,-1.));
#14646=DIRECTION('center_axis',(1.,0.,0.));
#14647=DIRECTION('ref_axis',(0.,0.,-1.));
#14648=DIRECTION('',(1.,0.,0.));
#14649=DIRECTION('center_axis',(1.,0.,0.));
#14650=DIRECTION('ref_axis',(0.,0.,-1.));
#14651=DIRECTION('',(0.,0.,-1.));
#14652=DIRECTION('center_axis',(0.,0.,1.));
#14653=DIRECTION('ref_axis',(1.,0.,0.));
#14654=DIRECTION('',(0.,1.,0.));
#14655=DIRECTION('center_axis',(0.,0.,1.));
#14656=DIRECTION('ref_axis',(1.,0.,0.));
#14657=DIRECTION('center_axis',(0.,0.,1.));
#14658=DIRECTION('ref_axis',(1.,0.,0.));
#14659=DIRECTION('center_axis',(0.,0.,-1.));
#14660=DIRECTION('ref_axis',(1.,0.,0.));
#14661=DIRECTION('',(0.,0.,-1.));
#14662=DIRECTION('center_axis',(0.,0.,-1.));
#14663=DIRECTION('ref_axis',(1.,0.,0.));
#14664=DIRECTION('center_axis',(0.,0.,1.));
#14665=DIRECTION('ref_axis',(1.,0.,0.));
#14666=DIRECTION('',(0.,0.,-1.));
#14667=DIRECTION('center_axis',(0.,0.,1.));
#14668=DIRECTION('ref_axis',(1.,0.,0.));
#14669=DIRECTION('center_axis',(0.,0.,1.));
#14670=DIRECTION('ref_axis',(1.,0.,0.));
#14671=DIRECTION('center_axis',(0.,1.,0.));
#14672=DIRECTION('ref_axis',(-1.,0.,0.));
#14673=DIRECTION('',(-1.,0.,0.));
#14674=DIRECTION('',(0.,0.,1.));
#14675=DIRECTION('center_axis',(1.,0.,0.));
#14676=DIRECTION('ref_axis',(0.,1.,0.));
#14677=DIRECTION('',(0.,1.,0.));
#14678=DIRECTION('',(0.,0.,1.));
#14679=DIRECTION('center_axis',(0.,-1.,0.));
#14680=DIRECTION('ref_axis',(1.,0.,0.));
#14681=DIRECTION('',(1.,0.,0.));
#14682=DIRECTION('center_axis',(0.,0.,1.));
#14683=DIRECTION('ref_axis',(1.,0.,0.));
#14684=DIRECTION('center_axis',(0.,0.,1.));
#14685=DIRECTION('ref_axis',(1.,0.,0.));
#18009=CARTESIAN_POINT('',(0.,0.,0.));
#18010=CARTESIAN_POINT('Origin',(2.4,-1.6,24.4));
#18011=CARTESIAN_POINT('',(2.235,-1.6,24.4));
#18012=CARTESIAN_POINT('Origin',(2.4,-1.6,24.4));
#18013=CARTESIAN_POINT('',(2.235,-1.6,25.));
#18014=CARTESIAN_POINT('',(2.235,-1.6,24.4));
#18015=CARTESIAN_POINT('Origin',(2.4,-1.6,25.));
#18016=CARTESIAN_POINT('Origin',(2.4,-1.6,24.4));
#18017=CARTESIAN_POINT('Origin',(2.4,1.6,24.4));
#18018=CARTESIAN_POINT('',(2.235,1.6,24.4));
#18019=CARTESIAN_POINT('Origin',(2.4,1.6,24.4));
#18020=CARTESIAN_POINT('',(2.235,1.6,25.));
#18021=CARTESIAN_POINT('',(2.235,1.6,24.4));
#18022=CARTESIAN_POINT('Origin',(2.4,1.6,25.));
#18023=CARTESIAN_POINT('Origin',(2.4,1.6,24.4));
#18024=CARTESIAN_POINT('Origin',(0.21,1.01,22.9));
#18025=CARTESIAN_POINT('',(-0.726238685697896,1.01,23.));
#18026=CARTESIAN_POINT('',(-0.726238685697896,1.01,25.));
#18027=CARTESIAN_POINT('',(-0.726238685697896,1.01,23.));
#18028=CARTESIAN_POINT('',(0.0305156009506911,1.01,23.));
#18029=CARTESIAN_POINT('',(1.98,1.01,23.));
#18030=CARTESIAN_POINT('',(0.0305156009506911,1.01,25.));
#18031=CARTESIAN_POINT('',(0.0305156009506911,1.01,22.9));
#18032=CARTESIAN_POINT('',(1.98,1.01,25.));
#18033=CARTESIAN_POINT('Origin',(-1.1,-1.01,22.9));
#18034=CARTESIAN_POINT('',(-0.726238685697896,-1.01,25.));
#18035=CARTESIAN_POINT('',(-0.726238685697896,-1.01,23.));
#18036=CARTESIAN_POINT('',(-0.726238685697896,-1.01,23.));
#18037=CARTESIAN_POINT('',(0.0305156009506911,-1.01,25.));
#18038=CARTESIAN_POINT('',(1.325,-1.01,25.));
#18039=CARTESIAN_POINT('',(0.0305156009506911,-1.01,23.));
#18040=CARTESIAN_POINT('',(0.0305156009506911,-1.01,22.9));
#18041=CARTESIAN_POINT('',(1.325,-1.01,23.));
#18042=CARTESIAN_POINT('Origin',(3.75,0.,23.));
#18043=CARTESIAN_POINT('',(1.,2.,23.));
#18044=CARTESIAN_POINT('Origin',(1.,0.,23.));
#18045=CARTESIAN_POINT('',(4.5,2.,23.));
#18046=CARTESIAN_POINT('',(6.5,2.,23.));
#18047=CARTESIAN_POINT('',(4.5,-2.,23.));
#18048=CARTESIAN_POINT('',(4.5,1.25,23.));
#18049=CARTESIAN_POINT('',(1.,-2.,23.));
#18050=CARTESIAN_POINT('',(1.,-2.,23.));
#18051=CARTESIAN_POINT('Origin',(1.,0.,23.));
#18052=CARTESIAN_POINT('Origin',(1.,0.,23.));
#18053=CARTESIAN_POINT('Origin',(1.,0.,22.9));
#18054=CARTESIAN_POINT('Origin',(1.,0.,25.));
#18055=CARTESIAN_POINT('Origin',(1.,0.,23.));
#18056=CARTESIAN_POINT('',(1.,-2.,25.));
#18057=CARTESIAN_POINT('',(1.,-2.,23.));
#18058=CARTESIAN_POINT('Origin',(1.,0.,25.));
#18059=CARTESIAN_POINT('Origin',(1.,0.,23.));
#18060=CARTESIAN_POINT('',(1.,2.,25.));
#18061=CARTESIAN_POINT('Origin',(1.,0.,25.));
#18062=CARTESIAN_POINT('',(1.,2.,23.));
#18063=CARTESIAN_POINT('Origin',(3.75,0.,25.));
#18064=CARTESIAN_POINT('',(4.5,-2.,25.));
#18065=CARTESIAN_POINT('',(1.,-2.,25.));
#18066=CARTESIAN_POINT('',(4.5,2.,25.));
#18067=CARTESIAN_POINT('',(4.5,1.25,25.));
#18068=CARTESIAN_POINT('',(6.5,2.,25.));
#18069=CARTESIAN_POINT('Origin',(1.,-2.,23.));
#18070=CARTESIAN_POINT('',(4.5,-2.,18.));
#18071=CARTESIAN_POINT('Origin',(6.5,2.,23.));
#18072=CARTESIAN_POINT('',(4.5,2.,18.));
#18073=CARTESIAN_POINT('Origin',(2.4,-1.6,14.4));
#18074=CARTESIAN_POINT('',(2.235,-1.6,14.4));
#18075=CARTESIAN_POINT('Origin',(2.4,-1.6,14.4));
#18076=CARTESIAN_POINT('',(2.235,-1.6,15.));
#18077=CARTESIAN_POINT('',(2.235,-1.6,14.4));
#18078=CARTESIAN_POINT('Origin',(2.4,-1.6,15.));
#18079=CARTESIAN_POINT('Origin',(2.4,-1.6,14.4));
#18080=CARTESIAN_POINT('Origin',(2.4,1.6,14.4));
#18081=CARTESIAN_POINT('',(2.235,1.6,14.4));
#18082=CARTESIAN_POINT('Origin',(2.4,1.6,14.4));
#18083=CARTESIAN_POINT('',(2.235,1.6,15.));
#18084=CARTESIAN_POINT('',(2.235,1.6,14.4));
#18085=CARTESIAN_POINT('Origin',(2.4,1.6,15.));
#18086=CARTESIAN_POINT('Origin',(2.4,1.6,14.4));
#18087=CARTESIAN_POINT('Origin',(0.21,1.01,12.9));
#18088=CARTESIAN_POINT('',(-0.726238685697896,1.01,13.));
#18089=CARTESIAN_POINT('',(-0.726238685697896,1.01,15.));
#18090=CARTESIAN_POINT('',(-0.726238685697896,1.01,13.));
#18091=CARTESIAN_POINT('',(0.0305156009506911,1.01,13.));
#18092=CARTESIAN_POINT('',(2.855,1.01,13.));
#18093=CARTESIAN_POINT('',(0.0305156009506911,1.01,15.));
#18094=CARTESIAN_POINT('',(0.0305156009506911,1.01,12.9));
#18095=CARTESIAN_POINT('',(1.98,1.01,15.));
#18096=CARTESIAN_POINT('Origin',(-1.1,-1.01,12.9));
#18097=CARTESIAN_POINT('',(-0.726238685697896,-1.01,15.));
#18098=CARTESIAN_POINT('',(-0.726238685697896,-1.01,13.));
#18099=CARTESIAN_POINT('',(-0.726238685697896,-1.01,13.));
#18100=CARTESIAN_POINT('',(0.0305156009506911,-1.01,15.));
#18101=CARTESIAN_POINT('',(1.325,-1.01,15.));
#18102=CARTESIAN_POINT('',(0.0305156009506911,-1.01,13.));
#18103=CARTESIAN_POINT('',(0.0305156009506911,-1.01,12.9));
#18104=CARTESIAN_POINT('',(2.2,-1.01,13.));
#18105=CARTESIAN_POINT('Origin',(5.5,0.,13.));
#18106=CARTESIAN_POINT('',(1.,2.,13.));
#18107=CARTESIAN_POINT('Origin',(1.,0.,13.));
#18108=CARTESIAN_POINT('',(4.5,2.,13.));
#18109=CARTESIAN_POINT('',(6.5,2.,13.));
#18110=CARTESIAN_POINT('',(4.5,2.5,13.));
#18111=CARTESIAN_POINT('',(4.5,2.5,13.));
#18112=CARTESIAN_POINT('',(6.5,2.5,13.));
#18113=CARTESIAN_POINT('',(6.5,2.5,13.));
#18114=CARTESIAN_POINT('',(6.5,0.979795897113272,13.));
#18115=CARTESIAN_POINT('',(6.5,-2.5,13.));
#18116=CARTESIAN_POINT('',(4.1,-1.71450551880629E-16,13.));
#18117=CARTESIAN_POINT('Origin',(5.5,0.,13.));
#18118=CARTESIAN_POINT('',(6.5,-0.979795897113272,13.));
#18119=CARTESIAN_POINT('Origin',(5.5,0.,13.));
#18120=CARTESIAN_POINT('',(6.5,-2.5,13.));
#18121=CARTESIAN_POINT('',(6.5,-2.5,13.));
#18122=CARTESIAN_POINT('',(4.5,-2.5,13.));
#18123=CARTESIAN_POINT('',(4.5,-2.5,13.));
#18124=CARTESIAN_POINT('',(4.5,-2.,13.));
#18125=CARTESIAN_POINT('',(4.5,2.5,13.));
#18126=CARTESIAN_POINT('',(1.,-2.,13.));
#18127=CARTESIAN_POINT('',(1.,-2.,13.));
#18128=CARTESIAN_POINT('Origin',(1.,0.,13.));
#18129=CARTESIAN_POINT('Origin',(1.,0.,13.));
#18130=CARTESIAN_POINT('Origin',(1.,0.,12.9));
#18131=CARTESIAN_POINT('Origin',(1.,0.,15.));
#18132=CARTESIAN_POINT('Origin',(1.,0.,13.));
#18133=CARTESIAN_POINT('',(1.,-2.,15.));
#18134=CARTESIAN_POINT('',(1.,-2.,13.));
#18135=CARTESIAN_POINT('Origin',(1.,0.,15.));
#18136=CARTESIAN_POINT('Origin',(1.,0.,13.));
#18137=CARTESIAN_POINT('',(1.,2.,15.));
#18138=CARTESIAN_POINT('Origin',(1.,0.,15.));
#18139=CARTESIAN_POINT('',(1.,2.,13.));
#18140=CARTESIAN_POINT('Origin',(3.75,0.,15.));
#18141=CARTESIAN_POINT('',(4.5,-2.,15.));
#18142=CARTESIAN_POINT('',(1.,-2.,15.));
#18143=CARTESIAN_POINT('',(4.5,2.,15.));
#18144=CARTESIAN_POINT('',(4.5,1.25,15.));
#18145=CARTESIAN_POINT('',(6.5,2.,15.));
#18146=CARTESIAN_POINT('Origin',(6.5,2.,13.));
#18147=CARTESIAN_POINT('',(4.5,2.,13.));
#18148=CARTESIAN_POINT('Origin',(1.,-2.,13.));
#18149=CARTESIAN_POINT('',(4.5,-2.,13.));
#18150=CARTESIAN_POINT('Origin',(4.5,2.5,13.));
#18151=CARTESIAN_POINT('',(4.5,-2.5,31.));
#18152=CARTESIAN_POINT('',(4.5,-2.5,13.));
#18153=CARTESIAN_POINT('',(4.5,2.5,31.));
#18154=CARTESIAN_POINT('',(4.5,2.5,31.));
#18155=CARTESIAN_POINT('',(4.5,2.5,13.));
#18156=CARTESIAN_POINT('Origin',(6.09,0.,12.2));
#18157=CARTESIAN_POINT('',(6.09,0.133884278389961,12.1035634923901));
#18158=CARTESIAN_POINT('',(6.09,0.133884278389961,12.2964365076099));
#18159=CARTESIAN_POINT('',(6.09,0.133884278389961,11.5));
#18160=CARTESIAN_POINT('Origin',(6.09,0.,12.2));
#18161=CARTESIAN_POINT('Origin',(6.09,0.,12.2));
#18162=CARTESIAN_POINT('',(6.09,-0.133884278389961,12.1035634923901));
#18163=CARTESIAN_POINT('Ctrl Pts',(6.09,-0.133884278389961,12.1035634923901));
#18164=CARTESIAN_POINT('Ctrl Pts',(6.09119840340611,-0.128603165341394,
12.0962316423768));
#18165=CARTESIAN_POINT('Ctrl Pts',(6.09244064128815,-0.122792448979944,
12.0894472111884));
#18166=CARTESIAN_POINT('Ctrl Pts',(6.09651064111414,-0.10208383195986,12.0687385941683));
#18167=CARTESIAN_POINT('Ctrl Pts',(6.09954409498317,-0.0836002135946602,
12.0560565239921));
#18168=CARTESIAN_POINT('Ctrl Pts',(6.10381707438298,-0.0429774150042655,
12.0391843843662));
#18169=CARTESIAN_POINT('Ctrl Pts',(6.105,-0.0208299403327841,12.035));
#18170=CARTESIAN_POINT('Ctrl Pts',(6.105,0.020829940332784,12.035));
#18171=CARTESIAN_POINT('Ctrl Pts',(6.10381707438298,0.0429774150042655,
12.0391843843662));
#18172=CARTESIAN_POINT('Ctrl Pts',(6.09954409498317,0.0836002135946602,
12.0560565239921));
#18173=CARTESIAN_POINT('Ctrl Pts',(6.09651064111414,0.10208383195986,12.0687385941683));
#18174=CARTESIAN_POINT('Ctrl Pts',(6.09244064128815,0.122792448979943,12.0894472111884));
#18175=CARTESIAN_POINT('Ctrl Pts',(6.09119840340611,0.128603165341395,12.0962316423768));
#18176=CARTESIAN_POINT('Ctrl Pts',(6.09,0.133884278389961,12.1035634923901));
#18177=CARTESIAN_POINT('',(6.09,-0.133884278389961,12.2964365076099));
#18178=CARTESIAN_POINT('Origin',(6.09,0.,12.2));
#18179=CARTESIAN_POINT('',(6.105,-2.74505708527337E-17,12.365));
#18180=CARTESIAN_POINT('Ctrl Pts',(6.105,1.11022302462516E-16,12.365));
#18181=CARTESIAN_POINT('Ctrl Pts',(6.105,-0.0208299403327839,12.365));
#18182=CARTESIAN_POINT('Ctrl Pts',(6.10381707438298,-0.0429774150042655,
12.3608156156338));
#18183=CARTESIAN_POINT('Ctrl Pts',(6.09954409498317,-0.0836002135946602,
12.3439434760079));
#18184=CARTESIAN_POINT('Ctrl Pts',(6.09651064111414,-0.10208383195986,12.3312614058317));
#18185=CARTESIAN_POINT('Ctrl Pts',(6.09244064128815,-0.122792448979944,
12.3105527888116));
#18186=CARTESIAN_POINT('Ctrl Pts',(6.09119840340611,-0.128603165341395,
12.3037683576232));
#18187=CARTESIAN_POINT('Ctrl Pts',(6.09,-0.133884278389961,12.2964365076099));
#18188=CARTESIAN_POINT('',(6.9,-2.02066721859312E-17,12.365));
#18189=CARTESIAN_POINT('',(6.09,-2.02066721859312E-17,12.365));
#18190=CARTESIAN_POINT('',(6.8902427845524,0.164999999999999,12.2));
#18191=CARTESIAN_POINT('Ctrl Pts',(6.8902427845524,0.164999999999999,12.2));
#18192=CARTESIAN_POINT('Ctrl Pts',(6.8902427845524,0.164999999999999,12.17926146026));
#18193=CARTESIAN_POINT('Ctrl Pts',(6.89075468722975,0.160851447474559,12.1571538860416));
#18194=CARTESIAN_POINT('Ctrl Pts',(6.89259968365095,0.144006627864299,12.1165070705051));
#18195=CARTESIAN_POINT('Ctrl Pts',(6.89390570229761,0.131311408395221,12.0979661706037));
#18196=CARTESIAN_POINT('Ctrl Pts',(6.89635413416378,0.102033925885227,12.0686886880937));
#18197=CARTESIAN_POINT('Ctrl Pts',(6.89765618378145,0.0834929839417266,
12.0559933930893));
#18198=CARTESIAN_POINT('Ctrl Pts',(6.89949208802221,0.042846026446055,12.0391485178689));
#18199=CARTESIAN_POINT('Ctrl Pts',(6.9,0.0207384030457212,12.035));
#18200=CARTESIAN_POINT('Ctrl Pts',(6.9,-0.0207384030457212,12.035));
#18201=CARTESIAN_POINT('Ctrl Pts',(6.89949208802221,-0.0428460264460565,
12.0391485178689));
#18202=CARTESIAN_POINT('Ctrl Pts',(6.89765618378145,-0.0834929839417278,
12.0559933930893));
#18203=CARTESIAN_POINT('Ctrl Pts',(6.89635413416378,-0.102033925885227,
12.0686886880937));
#18204=CARTESIAN_POINT('Ctrl Pts',(6.89390570229761,-0.131311408395221,
12.0979661706037));
#18205=CARTESIAN_POINT('Ctrl Pts',(6.89259968365095,-0.144006627864299,
12.1165070705051));
#18206=CARTESIAN_POINT('Ctrl Pts',(6.89075468722975,-0.160851447474559,
12.1571538860416));
#18207=CARTESIAN_POINT('Ctrl Pts',(6.8902427845524,-0.164999999999999,12.17926146026));
#18208=CARTESIAN_POINT('Ctrl Pts',(6.8902427845524,-0.164999999999999,12.22073853974));
#18209=CARTESIAN_POINT('Ctrl Pts',(6.89075468722975,-0.160851447474559,
12.2428461139584));
#18210=CARTESIAN_POINT('Ctrl Pts',(6.89259968365095,-0.144006627864299,
12.2834929294949));
#18211=CARTESIAN_POINT('Ctrl Pts',(6.89390570229761,-0.131311408395221,
12.3020338293963));
#18212=CARTESIAN_POINT('Ctrl Pts',(6.89635413416378,-0.102033925885227,
12.3313113119063));
#18213=CARTESIAN_POINT('Ctrl Pts',(6.89765618378145,-0.0834929839417278,
12.3440066069107));
#18214=CARTESIAN_POINT('Ctrl Pts',(6.89949208802221,-0.0428460264460565,
12.3608514821311));
#18215=CARTESIAN_POINT('Ctrl Pts',(6.9,-0.0207384030457213,12.365));
#18216=CARTESIAN_POINT('Ctrl Pts',(6.9,-1.14491749414469E-16,12.365));
#18217=CARTESIAN_POINT('Ctrl Pts',(6.9,6.93889390390723E-17,12.365));
#18218=CARTESIAN_POINT('Ctrl Pts',(6.9,0.0207384030457213,12.365));
#18219=CARTESIAN_POINT('Ctrl Pts',(6.89949208802221,0.0428460264460564,
12.3608514821311));
#18220=CARTESIAN_POINT('Ctrl Pts',(6.89765618378145,0.0834929839417278,
12.3440066069107));
#18221=CARTESIAN_POINT('Ctrl Pts',(6.89635413416378,0.102033925885227,12.3313113119063));
#18222=CARTESIAN_POINT('Ctrl Pts',(6.89390570229761,0.131311408395221,12.3020338293963));
#18223=CARTESIAN_POINT('Ctrl Pts',(6.89259968365095,0.144006627864299,12.2834929294949));
#18224=CARTESIAN_POINT('Ctrl Pts',(6.89075468722975,0.160851447474559,12.2428461139584));
#18225=CARTESIAN_POINT('Ctrl Pts',(6.8902427845524,0.164999999999999,12.22073853974));
#18226=CARTESIAN_POINT('Ctrl Pts',(6.8902427845524,0.164999999999999,12.2));
#18227=CARTESIAN_POINT('Ctrl Pts',(6.09,0.133884278389961,12.2964365076099));
#18228=CARTESIAN_POINT('Ctrl Pts',(6.09119840340611,0.128603165341395,12.3037683576232));
#18229=CARTESIAN_POINT('Ctrl Pts',(6.09244064128815,0.122792448979944,12.3105527888116));
#18230=CARTESIAN_POINT('Ctrl Pts',(6.09651064111414,0.10208383195986,12.3312614058317));
#18231=CARTESIAN_POINT('Ctrl Pts',(6.09954409498317,0.0836002135946602,
12.3439434760079));
#18232=CARTESIAN_POINT('Ctrl Pts',(6.10381707438298,0.0429774150042655,
12.3608156156338));
#18233=CARTESIAN_POINT('Ctrl Pts',(6.105,0.0208299403327841,12.365));
#18234=CARTESIAN_POINT('Ctrl Pts',(6.105,6.93889390390723E-17,12.365));
#18235=CARTESIAN_POINT('Origin',(6.09,0.,12.2));
#18236=CARTESIAN_POINT('',(6.09,-0.133884278389961,11.5));
#18237=CARTESIAN_POINT('Origin',(5.5,0.,13.));
#18238=CARTESIAN_POINT('',(6.5,-2.5,13.));
#18239=CARTESIAN_POINT('Origin',(5.5,0.,13.));
#18240=CARTESIAN_POINT('Origin',(5.5,0.,11.5));
#18241=CARTESIAN_POINT('',(4.895,-7.40911313484149E-17,13.));
#18242=CARTESIAN_POINT('Origin',(5.5,0.,13.));
#18243=CARTESIAN_POINT('',(4.895,-7.40911313484149E-17,11.5));
#18244=CARTESIAN_POINT('',(4.895,-7.40911313484149E-17,11.5));
#18245=CARTESIAN_POINT('Origin',(5.5,0.,11.5));
#18246=CARTESIAN_POINT('Origin',(5.5,0.,11.5));
#18247=CARTESIAN_POINT('',(4.1,-1.71450551880629E-16,11.5));
#18248=CARTESIAN_POINT('',(4.1,-1.71450551880629E-16,11.5));
#18249=CARTESIAN_POINT('Origin',(5.5,0.,11.5));
#18250=CARTESIAN_POINT('Origin',(5.5,0.,11.5));
#18251=CARTESIAN_POINT('Origin',(6.5,2.5,13.));
#18252=CARTESIAN_POINT('',(6.5,2.5,31.));
#18253=CARTESIAN_POINT('',(6.5,2.5,31.));
#18254=CARTESIAN_POINT('',(6.5,2.5,13.));
#18255=CARTESIAN_POINT('Origin',(6.5,-2.5,13.));
#18256=CARTESIAN_POINT('',(6.5,-2.5,31.));
#18257=CARTESIAN_POINT('',(6.5,-2.5,31.));
#18258=CARTESIAN_POINT('',(6.5,-2.5,13.));
#18259=CARTESIAN_POINT('Origin',(4.5,-2.5,13.));
#18260=CARTESIAN_POINT('',(4.5,-2.5,31.));
#18261=CARTESIAN_POINT('Origin',(5.5,0.,31.));
#18262=CARTESIAN_POINT('Origin',(5.5,0.,13.));
#33201=UNCERTAINTY_MEASURE_WITH_UNIT(LENGTH_MEASURE(0.001),#33300,
'DISTANCE_ACCURACY_VALUE',
'Maximum model space distance between geometric entities at asserted c
onnectivities');
#33247=UNCERTAINTY_MEASURE_WITH_UNIT(LENGTH_MEASURE(0.001),#33300,
'DISTANCE_ACCURACY_VALUE',
'Maximum model space distance between geometric entities at asserted c
onnectivities');
#33253=(
GEOMETRIC_REPRESENTATION_CONTEXT(3)
GLOBAL_UNCERTAINTY_ASSIGNED_CONTEXT((#33201))
GLOBAL_UNIT_ASSIGNED_CONTEXT((#33300,#33302,#33303))
REPRESENTATION_CONTEXT('','3D')
);
#33299=(
GEOMETRIC_REPRESENTATION_CONTEXT(3)
GLOBAL_UNCERTAINTY_ASSIGNED_CONTEXT((#33247))
GLOBAL_UNIT_ASSIGNED_CONTEXT((#33300,#33302,#33303))
REPRESENTATION_CONTEXT('','3D')
);
#33300=(
LENGTH_UNIT()
NAMED_UNIT(*)
SI_UNIT(.CENTI.,.METRE.)
);
#33302=(
NAMED_UNIT(*)
PLANE_ANGLE_UNIT()
SI_UNIT($,.RADIAN.)
);
#33303=(
NAMED_UNIT(*)
SI_UNIT($,.STERADIAN.)
SOLID_ANGLE_UNIT()
);
#33309=SHAPE_DEFINITION_REPRESENTATION(#33360,#33491);
#33360=PRODUCT_DEFINITION_SHAPE('',$,#33543);
#33491=SHAPE_REPRESENTATION('',(#13229),#33253);
#33537=PRODUCT_DEFINITION_CONTEXT('part definition',#33692,'design');
#33543=PRODUCT_DEFINITION('Head frame','Head frame',#33594,#33537);
#33594=PRODUCT_DEFINITION_FORMATION('',$,#33699);
#33692=APPLICATION_CONTEXT(
'Core Data for Automotive Mechanical Design Process');
#33693=PRODUCT_CONTEXT('part definition',#33692,'mechanical');
#33699=PRODUCT('Head frame','Head frame','Head frame',(#33693));
#33787=COLOUR_RGB('Dark Blue',0.08,0.2,0.34);
#33788=FILL_AREA_STYLE_COLOUR('',#33787);
#33789=FILL_AREA_STYLE('',(#33788));
#33790=SURFACE_STYLE_FILL_AREA(#33789);
#33791=SURFACE_SIDE_STYLE('',(#33790));
#33792=SURFACE_STYLE_USAGE(.BOTH.,#33791);
#33793=PRESENTATION_STYLE_ASSIGNMENT((#33792));
ENDSEC;
END-ISO-10303-21;
